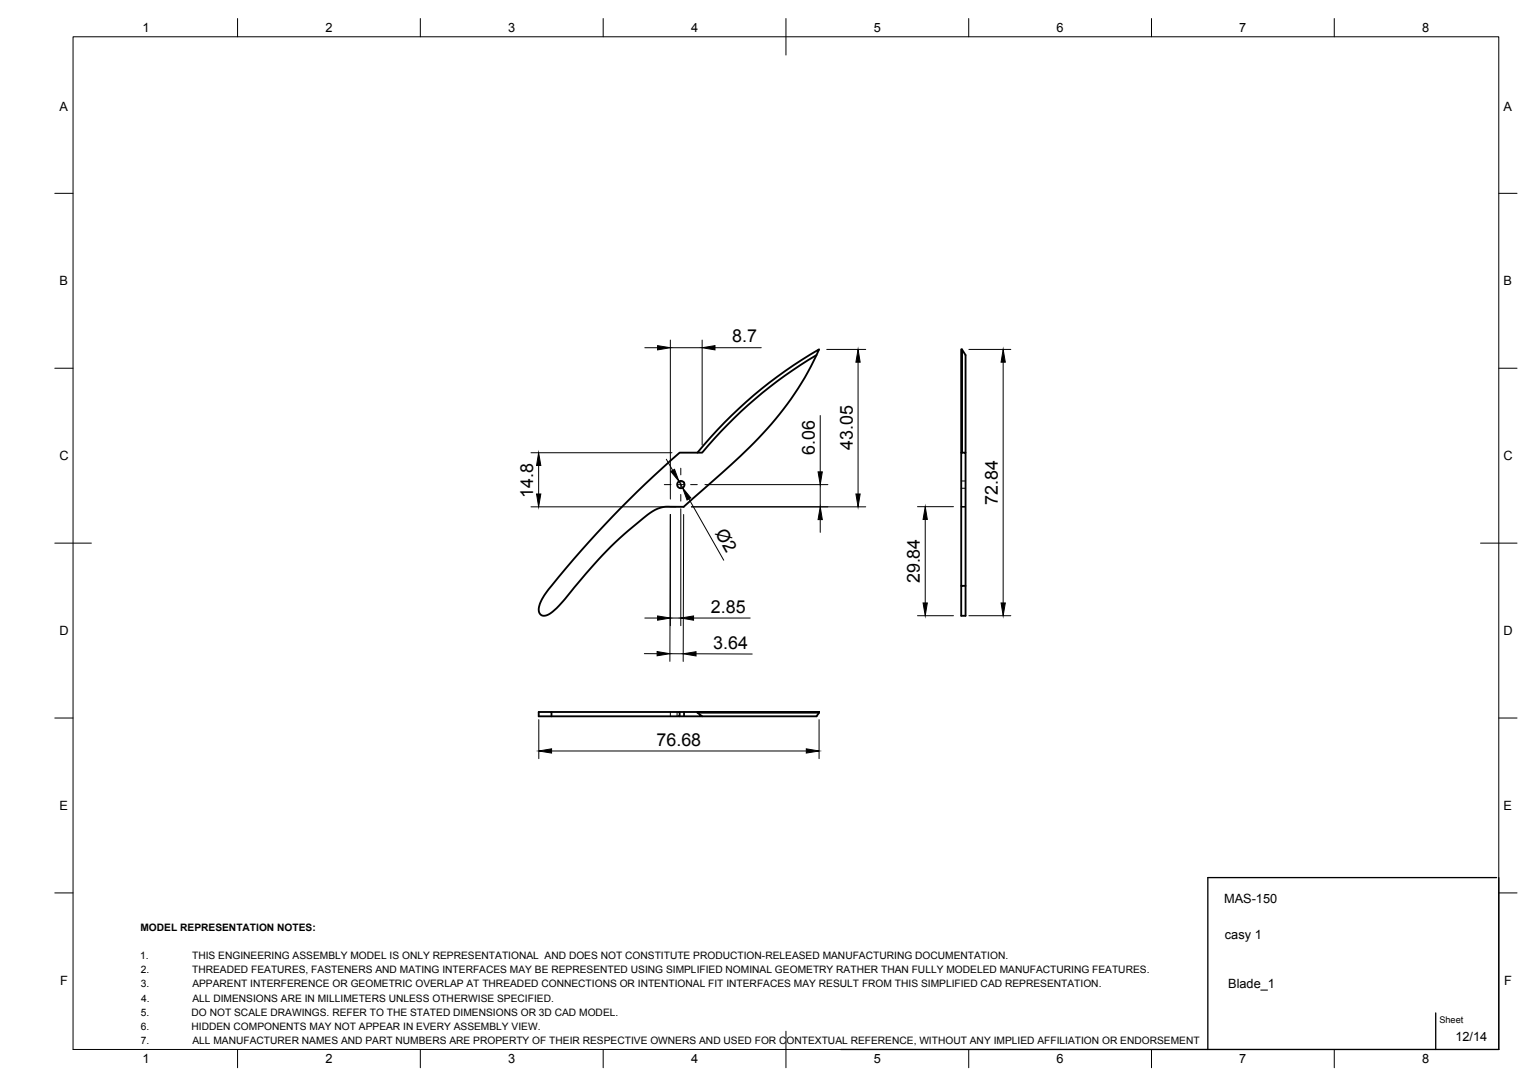
ISO-10303-21;
HEADER;
/* Generated by software containing ST-Developer
 * from STEP Tools, Inc. (www.steptools.com) 
 */

FILE_DESCRIPTION(
/* description */ ('STEP AP203'),
/* implementation_level */ '2;1');

FILE_NAME(
/* name */ 'Blade_1.step',
/* time_stamp */ '2026-11-08T21:40:52-08:00',
/* author */ (''),
/* organization */ (''),
/* preprocessor_version */ 'ST-DEVELOPER v20.2',
/* originating_system */ 'Autodesk Translation Framework v15.17.0.0',
/* authorisation */ '');

FILE_SCHEMA (('AUTOMOTIVE_DESIGN { 1 0 10303 214 3 1 1 }'));
ENDSEC;

DATA;
#10=MECHANICAL_DESIGN_GEOMETRIC_PRESENTATION_REPRESENTATION('',(#186),#12137);
#103=B_SPLINE_CURVE_WITH_KNOTS('',3,(#4610,#4611,#4612,#4613,#4614,#4615,
#4616,#4617,#4618,#4619,#4620,#4621,#4622,#4623,#4624,#4625,#4626,#4627,
#4628,#4629,#4630,#4631,#4632,#4633,#4634,#4635,#4636,#4637,#4638,#4639,
#4640,#4641,#4642,#4643,#4644,#4645,#4646,#4647,#4648,#4649,#4650,#4651,
#4652,#4653,#4654,#4655,#4656,#4657,#4658,#4659,#4660,#4661,#4662,#4663,
#4664,#4665),.UNSPECIFIED.,.F.,.F.,(4,2,2,2,2,1,2,2,2,2,2,2,2,2,2,2,2,2,
2,2,2,2,2,1,2,2,2,2,4),(1.76202838341362E-9,0.00152946839585409,0.00573422822705338,
0.00994072554036124,0.0183588914643831,0.0352156178566175,0.0520989766057049,
0.0859428491008545,0.153919387862698,0.222241646761829,0.256517065813169,
0.290860192348371,0.35972332278199,0.4287774185551,0.497967334131587,0.571128173595134,
0.636528988048645,0.709831201875327,0.774953293421917,0.843972576608793,
0.878409790177993,0.91278972931851,0.947105790641693,0.964237837412799,
0.981351495675405,0.989901182362907,0.994174197253835,0.998445976951636,
0.999999997793755),.UNSPECIFIED.);
#104=B_SPLINE_CURVE_WITH_KNOTS('',2,(#4668,#4669,#4670),.UNSPECIFIED.,.F.,
 .F.,(3,3),(0.,1.),.UNSPECIFIED.);
#105=B_SPLINE_CURVE_WITH_KNOTS('',3,(#4684,#4685,#4686,#4687,#4688,#4689,
#4690,#4691,#4692,#4693,#4694,#4695,#4696),.UNSPECIFIED.,.F.,.F.,(4,3,3,
3,4),(-0.197909908995898,-0.15516480831031,-0.111768121995836,-0.0989540665429965,
0.),.UNSPECIFIED.);
#106=B_SPLINE_CURVE_WITH_KNOTS('',3,(#4698,#4699,#4700,#4701,#4702),
 .UNSPECIFIED.,.F.,.F.,(4,1,4),(0.0298132943020683,0.494943232770503,1.),
 .UNSPECIFIED.);
#107=B_SPLINE_CURVE_WITH_KNOTS('',3,(#4705,#4706,#4707,#4708,#4709),
 .UNSPECIFIED.,.F.,.F.,(4,1,4),(0.,0.494943232770503,1.),.UNSPECIFIED.);
#108=B_SPLINE_CURVE_WITH_KNOTS('',3,(#4738,#4739,#4740,#4741,#4742,#4743,
#4744,#4745,#4746,#4747,#4748,#4749),.UNSPECIFIED.,.F.,.F.,(4,1,1,1,1,1,
1,1,1,4),(0.0654911701302355,0.0728325313021349,0.151642943092782,0.236641834545795,
0.351573197840935,0.540150564955284,0.71598472862448,0.797600110822501,
0.875509677594327,1.),.UNSPECIFIED.);
#109=B_SPLINE_CURVE_WITH_KNOTS('',3,(#4752,#4753,#4754,#4755,#4756,#4757,
#4758,#4759,#4760,#4761,#4762,#4763),.UNSPECIFIED.,.F.,.F.,(4,1,1,1,1,1,
1,1,1,4),(0.0654911701302355,0.0728325313021349,0.151642943092782,0.236641834545795,
0.351573197840935,0.540150564955284,0.71598472862448,0.797600110822501,
0.875509677594327,1.),.UNSPECIFIED.);
#110=B_SPLINE_CURVE_WITH_KNOTS('',2,(#4771,#4772,#4773),.UNSPECIFIED.,.F.,
 .F.,(3,3),(0.,1.),.UNSPECIFIED.);
#111=B_SPLINE_CURVE_WITH_KNOTS('',2,(#4776,#4777,#4778),.UNSPECIFIED.,.F.,
 .F.,(3,3),(0.,1.),.UNSPECIFIED.);
#112=B_SPLINE_CURVE_WITH_KNOTS('',3,(#4782,#4783,#4784,#4785,#4786,#4787),
 .UNSPECIFIED.,.F.,.F.,(4,2,4),(-0.229871652660954,-0.114908525875315,0.),
 .UNSPECIFIED.);
#113=B_SPLINE_CURVE_WITH_KNOTS('',3,(#4792,#4793,#4794,#4795,#4796,#4797,
#4798,#4799,#4800,#4801,#4802,#4803,#4804,#4805,#4806,#4807,#4808,#4809,
#4810,#4811,#4812,#4813,#4814,#4815,#4816,#4817,#4818,#4819,#4820,#4821,
#4822,#4823,#4824,#4825,#4826,#4827,#4828,#4829,#4830,#4831,#4832,#4833,
#4834,#4835,#4836,#4837,#4838,#4839,#4840,#4841,#4842,#4843,#4844,#4845,
#4846,#4847,#4848,#4849,#4850,#4851,#4852,#4853,#4854,#4855,#4856,#4857,
#4858),.UNSPECIFIED.,.F.,.F.,(4,3,3,3,3,3,3,3,3,3,3,3,3,3,3,3,3,3,3,3,3,
3,4),(-4.14191399419292,-4.12414475765899,-4.04926436109822,-3.89944091710028,
-3.74954461699361,-3.59958832872791,-3.29954750710329,-2.90481294303335,
-2.69931657063712,-2.30568273196656,-2.09957968336527,-2.07307122857376,
-2.04569728092775,-1.79983587858531,-1.49976903624527,-1.19950941255717,
-1.0493493530693,-0.899191607974707,-0.598950483849536,-0.298920557742038,
-0.149026588716908,-0.0741171167945361,-1.00000000280431E-6),
 .UNSPECIFIED.);
#147=B_SPLINE_SURFACE_WITH_KNOTS('',2,1,((#4600,#4601),(#4602,#4603),(#4604,
#4605)),.UNSPECIFIED.,.F.,.F.,.F.,(3,3),(2,2),(0.,1.),(0.,0.0287999999999918),
 .UNSPECIFIED.);
#148=B_SPLINE_SURFACE_WITH_KNOTS('',3,1,((#4671,#4672),(#4673,#4674),(#4675,
#4676),(#4677,#4678),(#4679,#4680),(#4681,#4682)),.UNSPECIFIED.,.F.,.F.,
 .F.,(4,1,1,4),(2,2),(0.,0.494943232770503,0.789351610361564,1.),(0.,0.17280000000419),
 .UNSPECIFIED.);
#149=B_SPLINE_SURFACE_WITH_KNOTS('',3,1,((#4710,#4711),(#4712,#4713),(#4714,
#4715),(#4716,#4717),(#4718,#4719),(#4720,#4721),(#4722,#4723),(#4724,#4725),
(#4726,#4727),(#4728,#4729),(#4730,#4731),(#4732,#4733)),.UNSPECIFIED.,
 .F.,.F.,.F.,(4,1,1,1,1,1,1,1,1,4),(2,2),(0.0654911701302355,0.0728325313021349,
0.151642943092782,0.236641834545795,0.351573197840935,0.540150564955284,
0.71598472862448,0.797600110822501,0.875509677594327,1.),(0.,0.1728),
 .UNSPECIFIED.);
#150=B_SPLINE_SURFACE_WITH_KNOTS('',2,1,((#4764,#4765),(#4766,#4767),(#4768,
#4769)),.UNSPECIFIED.,.F.,.F.,.F.,(3,3),(2,2),(0.,1.),(0.,0.1728),
 .UNSPECIFIED.);
#151=B_SPLINE_SURFACE_WITH_KNOTS('',1,3,((#4861,#4862,#4863,#4864,#4865,
#4866,#4867,#4868,#4869,#4870,#4871,#4872,#4873,#4874,#4875,#4876,#4877,
#4878,#4879,#4880,#4881,#4882,#4883,#4884,#4885,#4886,#4887,#4888,#4889,
#4890,#4891,#4892,#4893,#4894,#4895,#4896,#4897,#4898,#4899,#4900,#4901,
#4902,#4903,#4904,#4905,#4906,#4907,#4908,#4909,#4910,#4911,#4912,#4913,
#4914,#4915,#4916,#4917,#4918,#4919,#4920,#4921,#4922,#4923,#4924,#4925,
#4926,#4927,#4928,#4929,#4930,#4931,#4932,#4933,#4934,#4935,#4936,#4937,
#4938,#4939,#4940),(#4941,#4942,#4943,#4944,#4945,#4946,#4947,#4948,#4949,
#4950,#4951,#4952,#4953,#4954,#4955,#4956,#4957,#4958,#4959,#4960,#4961,
#4962,#4963,#4964,#4965,#4966,#4967,#4968,#4969,#4970,#4971,#4972,#4973,
#4974,#4975,#4976,#4977,#4978,#4979,#4980,#4981,#4982,#4983,#4984,#4985,
#4986,#4987,#4988,#4989,#4990,#4991,#4992,#4993,#4994,#4995,#4996,#4997,
#4998,#4999,#5000,#5001,#5002,#5003,#5004,#5005,#5006,#5007,#5008,#5009,
#5010,#5011,#5012,#5013,#5014,#5015,#5016,#5017,#5018,#5019,#5020)),
 .UNSPECIFIED.,.F.,.F.,.F.,(2,2),(4,2,2,2,2,2,2,2,2,2,2,2,2,2,2,2,2,2,2,
2,2,2,2,2,2,2,2,2,2,2,2,2,2,2,2,2,2,2,2,4),(0.,1.),(0.0438296453716767,
0.0445782836066419,0.0449526027241245,0.0453269218416071,0.0457012409590896,
0.0458884005178309,0.0459819802972016,0.0460755600765722,0.0462627196353135,
0.0464498791940548,0.0468241983115374,0.0475728365465026,0.0483214747814677,
0.049818751251398,0.0528133041912587,0.0558078571311194,0.0573051336010497,
0.05880241007098,0.0617969630108407,0.0647915159507014,0.067786068890562,
0.0737751747702833,0.0797642806500047,0.0827588335898653,0.0842561100597957,
0.085753386529726,0.0872506629996563,0.0879993012346215,0.0887479394695867,
0.0891222585870692,0.0893094181458105,0.0894965777045518,0.0895901574839225,
0.0896837372632931,0.0898708968220344,0.0900580563807757,0.090245215939517,
0.0906195350569996,0.0909938541744821,0.0917424924094473),.UNSPECIFIED.);
#164=SHAPE_REPRESENTATION_RELATIONSHIP('SRR','None',#12188,#175);
#175=ADVANCED_BREP_SHAPE_REPRESENTATION('',(#197),#12129);
#186=STYLED_ITEM('',(#12253),#197);
#197=MANIFOLD_SOLID_BREP('Body1',#1831);
#213=FACE_BOUND('',#648,.T.);
#214=FACE_BOUND('',#650,.T.);
#244=PLANE('',#2018);
#245=PLANE('',#2019);
#246=PLANE('',#2020);
#247=PLANE('',#2021);
#307=LINE('',#4598,#401);
#308=LINE('',#4608,#402);
#309=LINE('',#4667,#403);
#310=LINE('',#4704,#404);
#311=LINE('',#4736,#405);
#312=LINE('',#4751,#406);
#313=LINE('',#4775,#407);
#314=LINE('',#4781,#408);
#315=LINE('',#4788,#409);
#316=LINE('',#4790,#410);
#317=LINE('',#4859,#411);
#401=VECTOR('',#2303,1.);
#402=VECTOR('',#2306,1000.);
#403=VECTOR('',#2307,1000.);
#404=VECTOR('',#2308,1000.);
#405=VECTOR('',#2309,1000.);
#406=VECTOR('',#2310,1000.);
#407=VECTOR('',#2311,1000.);
#408=VECTOR('',#2314,10.);
#409=VECTOR('',#2315,10.);
#410=VECTOR('',#2318,1000.);
#411=VECTOR('',#2321,1000.);
#472=CYLINDRICAL_SURFACE('',#2015,1.);
#523=FACE_OUTER_BOUND('',#641,.T.);
#524=FACE_OUTER_BOUND('',#642,.T.);
#525=FACE_OUTER_BOUND('',#643,.T.);
#526=FACE_OUTER_BOUND('',#644,.T.);
#527=FACE_OUTER_BOUND('',#645,.T.);
#528=FACE_OUTER_BOUND('',#646,.T.);
#529=FACE_OUTER_BOUND('',#647,.T.);
#530=FACE_OUTER_BOUND('',#649,.T.);
#531=FACE_OUTER_BOUND('',#651,.T.);
#532=FACE_OUTER_BOUND('',#652,.T.);
#641=EDGE_LOOP('',(#1377,#1378,#1379,#1380));
#642=EDGE_LOOP('',(#1381,#1382,#1383,#1384));
#643=EDGE_LOOP('',(#1385,#1386,#1387,#1388,#1389));
#644=EDGE_LOOP('',(#1390,#1391,#1392,#1393));
#645=EDGE_LOOP('',(#1394,#1395,#1396,#1397));
#646=EDGE_LOOP('',(#1398,#1399,#1400,#1401,#1402));
#647=EDGE_LOOP('',(#1403,#1404,#1405,#1406,#1407,#1408));
#648=EDGE_LOOP('',(#1409));
#649=EDGE_LOOP('',(#1410,#1411,#1412,#1413,#1414,#1415));
#650=EDGE_LOOP('',(#1416));
#651=EDGE_LOOP('',(#1417,#1418,#1419,#1420));
#652=EDGE_LOOP('',(#1421,#1422,#1423,#1424));
#761=CIRCLE('',#2016,1.);
#762=CIRCLE('',#2017,1.);
#874=VERTEX_POINT('',#4595);
#875=VERTEX_POINT('',#4597);
#876=VERTEX_POINT('',#4606);
#877=VERTEX_POINT('',#4607);
#878=VERTEX_POINT('',#4609);
#879=VERTEX_POINT('',#4666);
#880=VERTEX_POINT('',#4683);
#881=VERTEX_POINT('',#4697);
#882=VERTEX_POINT('',#4703);
#883=VERTEX_POINT('',#4734);
#884=VERTEX_POINT('',#4735);
#885=VERTEX_POINT('',#4737);
#886=VERTEX_POINT('',#4750);
#887=VERTEX_POINT('',#4770);
#888=VERTEX_POINT('',#4774);
#889=VERTEX_POINT('',#4780);
#1058=EDGE_CURVE('',#874,#874,#761,.T.);
#1059=EDGE_CURVE('',#874,#875,#307,.T.);
#1060=EDGE_CURVE('',#875,#875,#762,.T.);
#1061=EDGE_CURVE('',#876,#877,#308,.T.);
#1062=EDGE_CURVE('',#877,#878,#103,.T.);
#1063=EDGE_CURVE('',#879,#878,#309,.T.);
#1064=EDGE_CURVE('',#876,#879,#104,.T.);
#1065=EDGE_CURVE('',#878,#880,#105,.T.);
#1066=EDGE_CURVE('',#880,#881,#106,.T.);
#1067=EDGE_CURVE('',#882,#881,#310,.T.);
#1068=EDGE_CURVE('',#879,#882,#107,.T.);
#1069=EDGE_CURVE('',#883,#884,#311,.T.);
#1070=EDGE_CURVE('',#885,#883,#108,.T.);
#1071=EDGE_CURVE('',#885,#886,#312,.T.);
#1072=EDGE_CURVE('',#886,#884,#109,.T.);
#1073=EDGE_CURVE('',#884,#887,#110,.T.);
#1074=EDGE_CURVE('',#888,#887,#313,.T.);
#1075=EDGE_CURVE('',#883,#888,#111,.T.);
#1076=EDGE_CURVE('',#887,#889,#314,.T.);
#1077=EDGE_CURVE('',#889,#877,#112,.T.);
#1078=EDGE_CURVE('',#888,#876,#315,.T.);
#1079=EDGE_CURVE('',#885,#882,#316,.T.);
#1080=EDGE_CURVE('',#880,#889,#113,.T.);
#1081=EDGE_CURVE('',#881,#886,#317,.T.);
#1377=ORIENTED_EDGE('',*,*,#1058,.F.);
#1378=ORIENTED_EDGE('',*,*,#1059,.T.);
#1379=ORIENTED_EDGE('',*,*,#1060,.T.);
#1380=ORIENTED_EDGE('',*,*,#1059,.F.);
#1381=ORIENTED_EDGE('',*,*,#1061,.T.);
#1382=ORIENTED_EDGE('',*,*,#1062,.T.);
#1383=ORIENTED_EDGE('',*,*,#1063,.F.);
#1384=ORIENTED_EDGE('',*,*,#1064,.F.);
#1385=ORIENTED_EDGE('',*,*,#1063,.T.);
#1386=ORIENTED_EDGE('',*,*,#1065,.T.);
#1387=ORIENTED_EDGE('',*,*,#1066,.T.);
#1388=ORIENTED_EDGE('',*,*,#1067,.F.);
#1389=ORIENTED_EDGE('',*,*,#1068,.F.);
#1390=ORIENTED_EDGE('',*,*,#1069,.F.);
#1391=ORIENTED_EDGE('',*,*,#1070,.F.);
#1392=ORIENTED_EDGE('',*,*,#1071,.T.);
#1393=ORIENTED_EDGE('',*,*,#1072,.T.);
#1394=ORIENTED_EDGE('',*,*,#1073,.T.);
#1395=ORIENTED_EDGE('',*,*,#1074,.F.);
#1396=ORIENTED_EDGE('',*,*,#1075,.F.);
#1397=ORIENTED_EDGE('',*,*,#1069,.T.);
#1398=ORIENTED_EDGE('',*,*,#1076,.T.);
#1399=ORIENTED_EDGE('',*,*,#1077,.T.);
#1400=ORIENTED_EDGE('',*,*,#1061,.F.);
#1401=ORIENTED_EDGE('',*,*,#1078,.F.);
#1402=ORIENTED_EDGE('',*,*,#1074,.T.);
#1403=ORIENTED_EDGE('',*,*,#1068,.T.);
#1404=ORIENTED_EDGE('',*,*,#1079,.F.);
#1405=ORIENTED_EDGE('',*,*,#1070,.T.);
#1406=ORIENTED_EDGE('',*,*,#1075,.T.);
#1407=ORIENTED_EDGE('',*,*,#1078,.T.);
#1408=ORIENTED_EDGE('',*,*,#1064,.T.);
#1409=ORIENTED_EDGE('',*,*,#1060,.F.);
#1410=ORIENTED_EDGE('',*,*,#1066,.F.);
#1411=ORIENTED_EDGE('',*,*,#1080,.T.);
#1412=ORIENTED_EDGE('',*,*,#1076,.F.);
#1413=ORIENTED_EDGE('',*,*,#1073,.F.);
#1414=ORIENTED_EDGE('',*,*,#1072,.F.);
#1415=ORIENTED_EDGE('',*,*,#1081,.F.);
#1416=ORIENTED_EDGE('',*,*,#1058,.T.);
#1417=ORIENTED_EDGE('',*,*,#1079,.T.);
#1418=ORIENTED_EDGE('',*,*,#1067,.T.);
#1419=ORIENTED_EDGE('',*,*,#1081,.T.);
#1420=ORIENTED_EDGE('',*,*,#1071,.F.);
#1421=ORIENTED_EDGE('',*,*,#1077,.F.);
#1422=ORIENTED_EDGE('',*,*,#1080,.F.);
#1423=ORIENTED_EDGE('',*,*,#1065,.F.);
#1424=ORIENTED_EDGE('',*,*,#1062,.F.);
#1751=ADVANCED_FACE('',(#523),#472,.F.);
#1752=ADVANCED_FACE('',(#524),#147,.F.);
#1753=ADVANCED_FACE('',(#525),#148,.F.);
#1754=ADVANCED_FACE('',(#526),#149,.F.);
#1755=ADVANCED_FACE('',(#527),#150,.F.);
#1756=ADVANCED_FACE('',(#528),#244,.F.);
#1757=ADVANCED_FACE('',(#529,#213),#245,.F.);
#1758=ADVANCED_FACE('',(#530,#214),#246,.T.);
#1759=ADVANCED_FACE('',(#531),#247,.F.);
#1760=ADVANCED_FACE('',(#532),#151,.T.);
#1831=CLOSED_SHELL('',(#1751,#1752,#1753,#1754,#1755,#1756,#1757,#1758,
#1759,#1760));
#2014=AXIS2_PLACEMENT_3D('',#4593,#2297,#2298);
#2015=AXIS2_PLACEMENT_3D('',#4594,#2299,#2300);
#2016=AXIS2_PLACEMENT_3D('',#4596,#2301,#2302);
#2017=AXIS2_PLACEMENT_3D('',#4599,#2304,#2305);
#2018=AXIS2_PLACEMENT_3D('',#4779,#2312,#2313);
#2019=AXIS2_PLACEMENT_3D('',#4789,#2316,#2317);
#2020=AXIS2_PLACEMENT_3D('',#4791,#2319,#2320);
#2021=AXIS2_PLACEMENT_3D('',#4860,#2322,#2323);
#2297=DIRECTION('axis',(0.,0.,1.));
#2298=DIRECTION('refdir',(1.,0.,0.));
#2299=DIRECTION('center_axis',(0.,1.,0.));
#2300=DIRECTION('ref_axis',(1.11022302462515E-16,0.,1.));
#2301=DIRECTION('center_axis',(0.,1.,0.));
#2302=DIRECTION('ref_axis',(1.11022302462515E-16,0.,1.));
#2303=DIRECTION('',(0.,1.,0.));
#2304=DIRECTION('center_axis',(0.,1.,0.));
#2305=DIRECTION('ref_axis',(1.11022302462515E-16,0.,1.));
#2306=DIRECTION('',(0.,-1.,0.));
#2307=DIRECTION('',(0.,-1.,0.));
#2308=DIRECTION('',(0.,-1.,0.));
#2309=DIRECTION('',(0.,-1.,0.));
#2310=DIRECTION('',(0.,-1.,0.));
#2311=DIRECTION('',(0.,-1.,0.));
#2312=DIRECTION('center_axis',(0.318513611714452,0.,0.94791828717069));
#2313=DIRECTION('ref_axis',(0.94791828717069,0.,-0.318513611714452));
#2314=DIRECTION('',(-0.94791828717069,0.,0.318513611714452));
#2315=DIRECTION('',(-0.947918287170691,0.,0.318513611714451));
#2316=DIRECTION('center_axis',(0.,-1.,0.));
#2317=DIRECTION('ref_axis',(-1.11022302462515E-16,0.,-1.));
#2318=DIRECTION('',(-0.946888830122557,0.,0.321561103663262));
#2319=DIRECTION('center_axis',(0.,-1.,0.));
#2320=DIRECTION('ref_axis',(-1.11022302462515E-16,0.,-1.));
#2321=DIRECTION('',(0.946888830122557,0.,-0.321561103663262));
#2322=DIRECTION('center_axis',(-0.321561103663262,0.,-0.946888830122557));
#2323=DIRECTION('ref_axis',(-0.946888830122557,0.,0.321561103663262));
#4593=CARTESIAN_POINT('',(0.,0.,0.));
#4594=CARTESIAN_POINT('Origin',(0.,0.,-0.451382872428838));
#4595=CARTESIAN_POINT('',(-2.33486982377251E-16,0.,-1.45138287242884));
#4596=CARTESIAN_POINT('Origin',(0.,0.,-0.451382872428838));
#4597=CARTESIAN_POINT('',(-2.33486982377251E-16,1.2,-1.45138287242884));
#4598=CARTESIAN_POINT('',(-2.3348698237725E-16,0.,-1.45138287242884));
#4599=CARTESIAN_POINT('Origin',(0.,1.2,-0.451382872428838));
#4600=CARTESIAN_POINT('Ctrl Pts',(-7.09134809128677,1.2,-7.28017474573539));
#4601=CARTESIAN_POINT('Ctrl Pts',(-7.09134809128677,0.912000000000082,-7.28017474573539));
#4602=CARTESIAN_POINT('Ctrl Pts',(-26.0573343465012,1.2,-19.1299473575062));
#4603=CARTESIAN_POINT('Ctrl Pts',(-26.0573343465012,0.912000000000082,-19.1299473575062));
#4604=CARTESIAN_POINT('Ctrl Pts',(-47.6352267379569,1.2,-23.4630266781973));
#4605=CARTESIAN_POINT('Ctrl Pts',(-47.6352267379569,0.912000000000082,-23.4630266781973));
#4606=CARTESIAN_POINT('',(-7.09134809128677,1.2,-7.28017474573539));
#4607=CARTESIAN_POINT('',(-7.09134823816015,1.00000000000006,-7.28017467283774));
#4608=CARTESIAN_POINT('',(-7.09134809128677,1.2,-7.28017474573539));
#4609=CARTESIAN_POINT('',(-47.6352266725888,1.00000007481202,-23.463026510487));
#4610=CARTESIAN_POINT('Ctrl Pts',(-7.09134831553042,1.00000000000006,-7.28017453553405));
#4611=CARTESIAN_POINT('Ctrl Pts',(-7.11068751337854,1.00000000000006,-7.29225607297566));
#4612=CARTESIAN_POINT('Ctrl Pts',(-7.13014127538947,1.00000000000006,-7.3044055075262));
#4613=CARTESIAN_POINT('Ctrl Pts',(-7.20288303224859,1.00000000000006,-7.34979888829056));
#4614=CARTESIAN_POINT('Ctrl Pts',(-7.2562856468552,1.00000000000006,-7.38307141655157));
#4615=CARTESIAN_POINT('Ctrl Pts',(-7.36308604485071,1.00000000000006,-7.44950314916467));
#4616=CARTESIAN_POINT('Ctrl Pts',(-7.41650933220709,1.00000000000006,-7.48267908965507));
#4617=CARTESIAN_POINT('Ctrl Pts',(-7.57688126501097,1.00000000000006,-7.58210746819504));
#4618=CARTESIAN_POINT('Ctrl Pts',(-7.68386634925554,1.00000000000006,-7.64821950621151));
#4619=CARTESIAN_POINT('Ctrl Pts',(-8.00522827087396,1.00000000000006,-7.84615547748184));
#4620=CARTESIAN_POINT('Ctrl Pts',(-8.43461654073609,1.00000000000006,-8.10888740557686));
#4621=CARTESIAN_POINT('Ctrl Pts',(-8.86481189078967,1.00000000000006,-8.36863733500345));
#4622=CARTESIAN_POINT('Ctrl Pts',(-9.51221899491459,1.00000000000005,-8.75693190854638));
#4623=CARTESIAN_POINT('Ctrl Pts',(-9.94498238629759,1.00000000000006,-9.01300707260298));
#4624=CARTESIAN_POINT('Ctrl Pts',(-11.2495773841444,1.00000000000006,-9.77452717708374));
#4625=CARTESIAN_POINT('Ctrl Pts',(-12.1240421591257,1.00000000000006,-10.2710077251322));
#4626=CARTESIAN_POINT('Ctrl Pts',(-13.8850801361361,1.00000000000006,-11.2430286125482));
#4627=CARTESIAN_POINT('Ctrl Pts',(-14.7716680498301,1.00000000000006,-11.7184360575102));
#4628=CARTESIAN_POINT('Ctrl Pts',(-16.1094164672201,1.00000000000006,-12.4149117109426));
#4629=CARTESIAN_POINT('Ctrl Pts',(-16.5574356159811,1.00000000000006,-12.6446827728682));
#4630=CARTESIAN_POINT('Ctrl Pts',(-17.4559246536095,1.00000000000006,-13.0985360950426));
#4631=CARTESIAN_POINT('Ctrl Pts',(-17.906495383924,1.00000000000006,-13.3226581958257));
#4632=CARTESIAN_POINT('Ctrl Pts',(-19.2630950583786,1.00000000000006,-13.9870499958456));
#4633=CARTESIAN_POINT('Ctrl Pts',(-20.1719150319432,1.00000000000006,-14.4182572383939));
#4634=CARTESIAN_POINT('Ctrl Pts',(-21.9998979114302,1.00000000000006,-15.2579388305516));
#4635=CARTESIAN_POINT('Ctrl Pts',(-22.9191119697774,1.00000000000006,-15.6663622503542));
#4636=CARTESIAN_POINT('Ctrl Pts',(-24.768006788053,1.00000000000006,-16.4603187472532));
#4637=CARTESIAN_POINT('Ctrl Pts',(-25.6976797513383,1.00000000000006,-16.8457952774682));
#4638=CARTESIAN_POINT('Ctrl Pts',(-27.620212900096,1.00000000000006,-17.6147290858774));
#4639=CARTESIAN_POINT('Ctrl Pts',(-28.6120762515168,1.00000000000006,-17.9961739561557));
#4640=CARTESIAN_POINT('Ctrl Pts',(-30.4984832918179,1.00000000000006,-18.6929702060858));
#4641=CARTESIAN_POINT('Ctrl Pts',(-31.3921908423818,1.00000000000006,-19.0110399067431));
#4642=CARTESIAN_POINT('Ctrl Pts',(-33.2952368599222,1.00000000000006,-19.6629165069278));
#4643=CARTESIAN_POINT('Ctrl Pts',(-34.3055473016782,1.00000000000006,-19.9939988746763));
#4644=CARTESIAN_POINT('Ctrl Pts',(-36.2228941614421,1.00000000000006,-20.5941180293612));
#4645=CARTESIAN_POINT('Ctrl Pts',(-37.1288738936713,1.00000000000006,-20.8659549929327));
#4646=CARTESIAN_POINT('Ctrl Pts',(-39.003851405174,1.00000000000006,-21.4044110917491));
#4647=CARTESIAN_POINT('Ctrl Pts',(-39.9735095225768,1.00000000000006,-21.6697762014278));
#4648=CARTESIAN_POINT('Ctrl Pts',(-41.4346591386383,1.00000000000006,-22.0500145741695));
#4649=CARTESIAN_POINT('Ctrl Pts',(-41.9223778391297,1.00000000000006,-22.1736882842118));
#4650=CARTESIAN_POINT('Ctrl Pts',(-42.8996532716617,1.00000000000006,-22.4150132014848));
#4651=CARTESIAN_POINT('Ctrl Pts',(-43.3893152843367,1.00000000000006,-22.5326978063825));
#4652=CARTESIAN_POINT('Ctrl Pts',(-44.3696193969244,1.00000000000006,-22.7618534517681));
#4653=CARTESIAN_POINT('Ctrl Pts',(-44.8604283639025,1.00000000000006,-22.8733785049591));
#4654=CARTESIAN_POINT('Ctrl Pts',(-45.5979342111895,1.00000000000006,-23.0361575203374));
#4655=CARTESIAN_POINT('Ctrl Pts',(-46.0894060993012,1.00000000000006,-23.1430409487816));
#4656=CARTESIAN_POINT('Ctrl Pts',(-46.5820249421721,1.00000000000006,-23.2469929425543));
#4657=CARTESIAN_POINT('Ctrl Pts',(-46.951626660381,1.00000000000006,-23.3237965794452));
#4658=CARTESIAN_POINT('Ctrl Pts',(-47.074831674522,1.00000000000006,-23.34920099103));
#4659=CARTESIAN_POINT('Ctrl Pts',(-47.2597235085411,1.00000000000006,-23.3870284915049));
#4660=CARTESIAN_POINT('Ctrl Pts',(-47.3213549739448,1.00000000000006,-23.3995884807167));
#4661=CARTESIAN_POINT('Ctrl Pts',(-47.4446371365223,1.00000000000006,-23.4246136938071));
#4662=CARTESIAN_POINT('Ctrl Pts',(-47.5063193313214,1.00000000000006,-23.4370845030402));
#4663=CARTESIAN_POINT('Ctrl Pts',(-47.5903801898929,1.00000000000006,-23.4540147689754));
#4664=CARTESIAN_POINT('Ctrl Pts',(-47.6128719552537,1.00000000000006,-23.4585359892155));
#4665=CARTESIAN_POINT('Ctrl Pts',(-47.6352267041176,1.00000000000006,-23.4630263535246));
#4666=CARTESIAN_POINT('',(-47.6352267379569,1.2,-23.4630266781973));
#4667=CARTESIAN_POINT('',(-47.6352267379569,1.2,-23.4630266781973));
#4668=CARTESIAN_POINT('Ctrl Pts',(-7.09134809128677,1.2,-7.28017474573539));
#4669=CARTESIAN_POINT('Ctrl Pts',(-26.0573343465012,1.2,-19.1299473575062));
#4670=CARTESIAN_POINT('Ctrl Pts',(-47.6352267379569,1.2,-23.4630266781973));
#4671=CARTESIAN_POINT('Ctrl Pts',(-47.6352267379569,1.2,-23.4630266781973));
#4672=CARTESIAN_POINT('Ctrl Pts',(-47.6352267379569,-0.5280000000419,-23.4630266781973));
#4673=CARTESIAN_POINT('Ctrl Pts',(-41.2879795894165,1.2,-16.3973366595173));
#4674=CARTESIAN_POINT('Ctrl Pts',(-41.2879795894165,-0.5280000000419,-16.3973366595173));
#4675=CARTESIAN_POINT('Ctrl Pts',(-28.9390638541746,1.2,-7.40052527015664));
#4676=CARTESIAN_POINT('Ctrl Pts',(-28.9390638541746,-0.5280000000419,-7.40052527015664));
#4677=CARTESIAN_POINT('Ctrl Pts',(-11.4361348672924,1.2,0.292821829763132));
#4678=CARTESIAN_POINT('Ctrl Pts',(-11.4361348672924,-0.5280000000419,0.292821829763132));
#4679=CARTESIAN_POINT('Ctrl Pts',(-2.50014102937161,1.2,3.94559933269074));
#4680=CARTESIAN_POINT('Ctrl Pts',(-2.50014102937161,-0.5280000000419,3.94559933269074));
#4681=CARTESIAN_POINT('Ctrl Pts',(1.18077271965353,1.2,5.54861712757117));
#4682=CARTESIAN_POINT('Ctrl Pts',(1.18077271965353,-0.5280000000419,5.54861712757117));
#4683=CARTESIAN_POINT('',(-46.4732177923012,0.,-22.2016498092846));
#4684=CARTESIAN_POINT('Ctrl Pts',(-47.6352265853192,1.00000017512283,-23.4630265082826));
#4685=CARTESIAN_POINT('Ctrl Pts',(-47.5497337833158,0.923530724722877,-23.3678568040681));
#4686=CARTESIAN_POINT('Ctrl Pts',(-47.4664431491314,0.849654487371893,-23.275672245252));
#4687=CARTESIAN_POINT('Ctrl Pts',(-47.3838551040137,0.777007709588356,-23.1847477783321));
#4688=CARTESIAN_POINT('Ctrl Pts',(-47.3000081267036,0.7032535394808,-23.0924373028402));
#4689=CARTESIAN_POINT('Ctrl Pts',(-47.2168852312997,0.630766597197125,-23.0014256885189));
#4690=CARTESIAN_POINT('Ctrl Pts',(-47.1328800183873,0.558119808566171,-22.9099457634324));
#4691=CARTESIAN_POINT('Ctrl Pts',(-47.1080751876962,0.536668862490658,-22.8829338200692));
#4692=CARTESIAN_POINT('Ctrl Pts',(-47.0831931883918,0.515203979624482,-22.8558812926668));
#4693=CARTESIAN_POINT('Ctrl Pts',(-47.0581920598092,0.493688420180458,-22.8287433089684));
#4694=CARTESIAN_POINT('Ctrl Pts',(-46.8651256765308,0.327538670886058,-22.6191754750683));
#4695=CARTESIAN_POINT('Ctrl Pts',(-46.6701360902887,0.162956146341853,-22.4101382936785));
#4696=CARTESIAN_POINT('Ctrl Pts',(-46.4732177923012,0.,-22.2016498092846));
#4697=CARTESIAN_POINT('',(1.18077271965353,0.,5.54861712757117));
#4698=CARTESIAN_POINT('Ctrl Pts',(-46.4732177923012,0.,-22.2016498092846));
#4699=CARTESIAN_POINT('Ctrl Pts',(-40.3530658599041,0.,-15.7219005239919));
#4700=CARTESIAN_POINT('Ctrl Pts',(-25.1069939231375,0.,-4.7997213617563));
#4701=CARTESIAN_POINT('Ctrl Pts',(-7.64469421946831,0.,1.70517457060066));
#4702=CARTESIAN_POINT('Ctrl Pts',(1.18077271965353,0.,5.54861712757117));
#4703=CARTESIAN_POINT('',(1.18077271965353,1.2,5.54861712757117));
#4704=CARTESIAN_POINT('',(1.18077271965353,1.2,5.54861712757117));
#4705=CARTESIAN_POINT('Ctrl Pts',(-47.6352267379569,1.2,-23.4630266781973));
#4706=CARTESIAN_POINT('Ctrl Pts',(-41.2879795894165,1.2,-16.3973366595173));
#4707=CARTESIAN_POINT('Ctrl Pts',(-25.6436006166727,1.2,-4.99961317195811));
#4708=CARTESIAN_POINT('Ctrl Pts',(-7.64469421946831,1.2,1.70517457060066));
#4709=CARTESIAN_POINT('Ctrl Pts',(1.18077271965353,1.2,5.54861712757117));
#4710=CARTESIAN_POINT('Ctrl Pts',(4.63072594339218,1.2,4.37702154953648));
#4711=CARTESIAN_POINT('Ctrl Pts',(4.63072594339218,-0.528,4.37702154953648));
#4712=CARTESIAN_POINT('Ctrl Pts',(4.7840847941358,1.2,4.31192383490808));
#4713=CARTESIAN_POINT('Ctrl Pts',(4.7840847941358,-0.528,4.31192383490808));
#4714=CARTESIAN_POINT('Ctrl Pts',(6.57703737715603,1.2,3.59239489692552));
#4715=CARTESIAN_POINT('Ctrl Pts',(6.57703737715603,-0.528,3.59239489692552));
#4716=CARTESIAN_POINT('Ctrl Pts',(9.67706435206833,1.2,3.76607425470487));
#4717=CARTESIAN_POINT('Ctrl Pts',(9.67706435206833,-0.528,3.76607425470487));
#4718=CARTESIAN_POINT('Ctrl Pts',(14.6739773919611,1.2,5.78899007926008));
#4719=CARTESIAN_POINT('Ctrl Pts',(14.6739773919611,-0.528,5.78899007926008));
#4720=CARTESIAN_POINT('Ctrl Pts',(21.529136784602,1.2,8.35971201308491));
#4721=CARTESIAN_POINT('Ctrl Pts',(21.529136784602,-0.528,8.35971201308491));
#4722=CARTESIAN_POINT('Ctrl Pts',(29.5112752479747,1.2,12.6039811673409));
#4723=CARTESIAN_POINT('Ctrl Pts',(29.5112752479747,-0.528,12.6039811673409));
#4724=CARTESIAN_POINT('Ctrl Pts',(36.9335047542113,1.2,17.1028493432964));
#4725=CARTESIAN_POINT('Ctrl Pts',(36.9335047542113,-0.528,17.1028493432964));
#4726=CARTESIAN_POINT('Ctrl Pts',(41.8538494170237,1.2,20.3434433890621));
#4727=CARTESIAN_POINT('Ctrl Pts',(41.8538494170237,-0.528,20.3434433890621));
#4728=CARTESIAN_POINT('Ctrl Pts',(48.2654669907203,1.2,23.135880733102));
#4729=CARTESIAN_POINT('Ctrl Pts',(48.2654669907203,-0.528,23.135880733102));
#4730=CARTESIAN_POINT('Ctrl Pts',(48.9333109271159,1.2,18.4504184980571));
#4731=CARTESIAN_POINT('Ctrl Pts',(48.9333109271159,-0.528,18.4504184980571));
#4732=CARTESIAN_POINT('Ctrl Pts',(42.3375494192901,1.2,14.5257061310277));
#4733=CARTESIAN_POINT('Ctrl Pts',(42.3375494192901,-0.528,14.5257061310277));
#4734=CARTESIAN_POINT('',(42.3375494192901,1.2,14.5257061310277));
#4735=CARTESIAN_POINT('',(42.3375494192901,0.,14.5257061310277));
#4736=CARTESIAN_POINT('',(42.3375494192901,1.2,14.5257061310277));
#4737=CARTESIAN_POINT('',(4.63072594277028,1.2,4.37702154980046));
#4738=CARTESIAN_POINT('Ctrl Pts',(4.63072594339218,1.2,4.37702154953648));
#4739=CARTESIAN_POINT('Ctrl Pts',(4.7840847941358,1.2,4.31192383490808));
#4740=CARTESIAN_POINT('Ctrl Pts',(6.57703737715603,1.2,3.59239489692552));
#4741=CARTESIAN_POINT('Ctrl Pts',(9.67706435206833,1.2,3.76607425470487));
#4742=CARTESIAN_POINT('Ctrl Pts',(14.6739773919611,1.2,5.78899007926008));
#4743=CARTESIAN_POINT('Ctrl Pts',(21.529136784602,1.2,8.35971201308491));
#4744=CARTESIAN_POINT('Ctrl Pts',(29.5112752479747,1.2,12.6039811673409));
#4745=CARTESIAN_POINT('Ctrl Pts',(36.9335047542113,1.2,17.1028493432964));
#4746=CARTESIAN_POINT('Ctrl Pts',(41.8538494170237,1.2,20.3434433890621));
#4747=CARTESIAN_POINT('Ctrl Pts',(48.2654669907203,1.2,23.135880733102));
#4748=CARTESIAN_POINT('Ctrl Pts',(48.9333109271159,1.2,18.4504184980571));
#4749=CARTESIAN_POINT('Ctrl Pts',(42.3375494192901,1.2,14.5257061310277));
#4750=CARTESIAN_POINT('',(4.63072594277028,0.,4.37702154980046));
#4751=CARTESIAN_POINT('',(4.63072594277027,1.2,4.37702154980048));
#4752=CARTESIAN_POINT('Ctrl Pts',(4.63072594339218,4.16333634234434E-16,
4.37702154953648));
#4753=CARTESIAN_POINT('Ctrl Pts',(4.7840847941358,4.16333634234434E-16,
4.31192383490808));
#4754=CARTESIAN_POINT('Ctrl Pts',(6.57703737715603,4.16333634234434E-16,
3.59239489692552));
#4755=CARTESIAN_POINT('Ctrl Pts',(9.67706435206833,4.16333634234434E-16,
3.76607425470487));
#4756=CARTESIAN_POINT('Ctrl Pts',(14.6739773919611,4.16333634234434E-16,
5.78899007926008));
#4757=CARTESIAN_POINT('Ctrl Pts',(21.529136784602,4.16333634234434E-16,
8.35971201308491));
#4758=CARTESIAN_POINT('Ctrl Pts',(29.5112752479747,4.16333634234434E-16,
12.6039811673409));
#4759=CARTESIAN_POINT('Ctrl Pts',(36.9335047542113,4.16333634234434E-16,
17.1028493432964));
#4760=CARTESIAN_POINT('Ctrl Pts',(41.8538494170237,4.16333634234434E-16,
20.3434433890621));
#4761=CARTESIAN_POINT('Ctrl Pts',(48.2654669907203,4.16333634234434E-16,
23.135880733102));
#4762=CARTESIAN_POINT('Ctrl Pts',(48.9333109271159,4.16333634234434E-16,
18.4504184980571));
#4763=CARTESIAN_POINT('Ctrl Pts',(42.3375494192901,4.16333634234434E-16,
14.5257061310277));
#4764=CARTESIAN_POINT('Ctrl Pts',(42.3375494192901,1.2,14.5257061310277));
#4765=CARTESIAN_POINT('Ctrl Pts',(42.3375494192901,-0.528,14.5257061310277));
#4766=CARTESIAN_POINT('Ctrl Pts',(20.9640318338388,1.2,0.869135776253969));
#4767=CARTESIAN_POINT('Ctrl Pts',(20.9640318338388,-0.528,0.869135776253969));
#4768=CARTESIAN_POINT('Ctrl Pts',(-2.47626210225015,1.2,-8.83090725784708));
#4769=CARTESIAN_POINT('Ctrl Pts',(-2.47626210225015,-0.528,-8.83090725784708));
#4770=CARTESIAN_POINT('',(-2.47626210225015,0.,-8.83090725784708));
#4771=CARTESIAN_POINT('Ctrl Pts',(42.3375494192901,0.,14.5257061310277));
#4772=CARTESIAN_POINT('Ctrl Pts',(20.9640318338388,0.,0.869135776253969));
#4773=CARTESIAN_POINT('Ctrl Pts',(-2.47626210225015,0.,-8.83090725784708));
#4774=CARTESIAN_POINT('',(-2.47626210225015,1.2,-8.83090725784708));
#4775=CARTESIAN_POINT('',(-2.47626210225015,1.2,-8.83090725784708));
#4776=CARTESIAN_POINT('Ctrl Pts',(42.3375494192901,1.2,14.5257061310277));
#4777=CARTESIAN_POINT('Ctrl Pts',(20.9640318338388,1.2,0.869135776253969));
#4778=CARTESIAN_POINT('Ctrl Pts',(-2.47626210225015,1.2,-8.83090725784708));
#4779=CARTESIAN_POINT('Origin',(-2.47626210225015,1.2,-8.83090725784708));
#4780=CARTESIAN_POINT('',(-8.32185266851751,0.,-6.86670824505761));
#4781=CARTESIAN_POINT('',(-2.47626210225015,0.,-8.83090725784708));
#4782=CARTESIAN_POINT('Ctrl Pts',(-8.32185266851834,1.14311338172968E-12,
-6.86670824505734));
#4783=CARTESIAN_POINT('Ctrl Pts',(-8.11928072190117,0.164182972460768,-6.93477521161165));
#4784=CARTESIAN_POINT('Ctrl Pts',(-7.91680514284801,0.328508227719272,-7.00280979716715));
#4785=CARTESIAN_POINT('Ctrl Pts',(-7.51215815602449,0.657345458539218,-7.13877676287178));
#4786=CARTESIAN_POINT('Ctrl Pts',(-7.37869817804401,0.765866874721603,-7.18362115541202));
#4787=CARTESIAN_POINT('Ctrl Pts',(-7.09134844131163,1.00000001188238,-7.28017462812221));
#4788=CARTESIAN_POINT('',(-2.47626210225015,1.2,-8.83090725784708));
#4789=CARTESIAN_POINT('Origin',(-26.7103108805615,1.2,-17.2507740347362));
#4790=CARTESIAN_POINT('',(1.18077271965353,1.2,5.54861712757117));
#4791=CARTESIAN_POINT('Origin',(-26.7103108805615,0.,-17.2507740347362));
#4792=CARTESIAN_POINT('Ctrl Pts',(-46.4732177922936,0.,-22.2016498093203));
#4793=CARTESIAN_POINT('Ctrl Pts',(-46.415282761538,5.07841822769624E-16,
-22.1893264214989));
#4794=CARTESIAN_POINT('Ctrl Pts',(-46.3573586444288,1.28814513242496E-15,
-22.176961010912));
#4795=CARTESIAN_POINT('Ctrl Pts',(-46.2994454089906,1.77635683940025E-15,
-22.1645535547065));
#4796=CARTESIAN_POINT('Ctrl Pts',(-46.0553963173232,3.8337038815267E-15,
-22.1122679520467));
#4797=CARTESIAN_POINT('Ctrl Pts',(-45.8115404634548,5.56211880942695E-15,
-22.0592357000739));
#4798=CARTESIAN_POINT('Ctrl Pts',(-45.5678754638484,7.32747196252603E-15,
-22.0054550434754));
#4799=CARTESIAN_POINT('Ctrl Pts',(-45.0803415951789,1.08596553031322E-14,
-21.8978487331172));
#4800=CARTESIAN_POINT('Ctrl Pts',(-44.5935547144433,1.37433652042168E-14,
-21.7872420837894));
#4801=CARTESIAN_POINT('Ctrl Pts',(-44.1075470623437,1.62092561595273E-14,
-21.6736330559672));
#4802=CARTESIAN_POINT('Ctrl Pts',(-43.6213030745586,1.86763462277054E-14,
-21.559968782374));
#4803=CARTESIAN_POINT('Ctrl Pts',(-43.1356693881152,2.06773659315811E-14,
-21.443256509246));
#4804=CARTESIAN_POINT('Ctrl Pts',(-42.65115708627,2.26485497023532E-14,
-21.3236127657438));
#4805=CARTESIAN_POINT('Ctrl Pts',(-42.1664508837015,2.46205223363956E-14,
-21.2039211410871));
#4806=CARTESIAN_POINT('Ctrl Pts',(-41.6827582533232,2.48053267803675E-14,
-21.0812721899324));
#4807=CARTESIAN_POINT('Ctrl Pts',(-41.2001345714453,2.62012633811537E-14,
-20.9556779035789));
#4808=CARTESIAN_POINT('Ctrl Pts',(-40.2344744599496,2.87722289092885E-14,
-20.7043819205649));
#4809=CARTESIAN_POINT('Ctrl Pts',(-39.2727950142657,2.70692054571062E-14,
-20.4412269998355));
#4810=CARTESIAN_POINT('Ctrl Pts',(-38.3151477577178,2.62012633811537E-14,
-20.1662098332526));
#4811=CARTESIAN_POINT('Ctrl Pts',(-37.0552642848644,2.50593963007545E-14,
-19.8043964614086));
#4812=CARTESIAN_POINT('Ctrl Pts',(-35.8021293334856,2.23739275243883E-14,
-19.4219998183265));
#4813=CARTESIAN_POINT('Ctrl Pts',(-34.5554354702551,1.95399252334028E-14,
-19.018867339076));
#4814=CARTESIAN_POINT('Ctrl Pts',(-33.9064143565704,1.80645611706375E-14,
-18.8089990639827));
#4815=CARTESIAN_POINT('Ctrl Pts',(-33.2591391506989,1.64907532665174E-14,
-18.5935101896125));
#4816=CARTESIAN_POINT('Ctrl Pts',(-32.6135681765606,1.50990331349021E-14,
-18.3723738593228));
#4817=CARTESIAN_POINT('Ctrl Pts',(-31.3769595799164,1.24331557212291E-14,
-17.94878125987));
#4818=CARTESIAN_POINT('Ctrl Pts',(-30.1465313472377,1.0222160868584E-14,
-17.504445383288));
#4819=CARTESIAN_POINT('Ctrl Pts',(-28.9220387964689,9.76996261670138E-15,
-17.0391634027186));
#4820=CARTESIAN_POINT('Ctrl Pts',(-28.280905786778,9.53319578130951E-15,
-16.7955460476191));
#4821=CARTESIAN_POINT('Ctrl Pts',(-27.6414002959298,9.73942422296218E-15,
-16.5461855556373));
#4822=CARTESIAN_POINT('Ctrl Pts',(-27.003489002828,1.06581410364015E-14,
-16.2910473999339));
#4823=CARTESIAN_POINT('Ctrl Pts',(-26.9214424596597,1.07763040780476E-14,
-16.2582321732211));
#4824=CARTESIAN_POINT('Ctrl Pts',(-26.8394331456511,1.09599753714691E-14,
-16.2253257263837));
#4825=CARTESIAN_POINT('Ctrl Pts',(-26.7574608858174,1.11022302462516E-14,
-16.1923280234092));
#4826=CARTESIAN_POINT('Ctrl Pts',(-26.6728122570399,1.1249129698721E-14,
-16.158252955633));
#4827=CARTESIAN_POINT('Ctrl Pts',(-26.5882109329397,1.1627230561039E-14,
-16.1240837088094));
#4828=CARTESIAN_POINT('Ctrl Pts',(-26.5036601420706,1.17683640610267E-14,
-16.0898217001875));
#4829=CARTESIAN_POINT('Ctrl Pts',(-25.7442601358659,1.3035966405898E-14,
-15.7820946015686));
#4830=CARTESIAN_POINT('Ctrl Pts',(-24.9888454631677,1.38814835013908E-14,
-15.4668487724091));
#4831=CARTESIAN_POINT('Ctrl Pts',(-24.237230782582,1.46549439250521E-14,
-15.1440887362585));
#4832=CARTESIAN_POINT('Ctrl Pts',(-23.3199064620055,1.55989303531444E-14,
-14.7501693005172));
#4833=CARTESIAN_POINT('Ctrl Pts',(-22.4082668273739,1.50548750441534E-14,
-14.3450675510963));
#4834=CARTESIAN_POINT('Ctrl Pts',(-21.5020580029957,1.62092561595273E-14,
-13.9288016897425));
#4835=CARTESIAN_POINT('Ctrl Pts',(-20.5952669744745,1.73643789201489E-14,
-13.5122683936621));
#4836=CARTESIAN_POINT('Ctrl Pts',(-19.6938847201665,1.57933555484948E-14,
-13.0845414602457));
#4837=CARTESIAN_POINT('Ctrl Pts',(-18.7977536862311,1.62092561595273E-14,
-12.645663195712));
#4838=CARTESIAN_POINT('Ctrl Pts',(-18.3495978945471,1.63062227585341E-14,
-12.4261798515952));
#4839=CARTESIAN_POINT('Ctrl Pts',(-17.9027032335625,1.57814290351876E-14,
-12.2038797705404));
#4840=CARTESIAN_POINT('Ctrl Pts',(-17.4571099588515,1.55431223447522E-14,
-11.9787974606056));
#4841=CARTESIAN_POINT('Ctrl Pts',(-17.0115235519992,1.53048193273002E-14,
-11.7537186198289));
#4842=CARTESIAN_POINT('Ctrl Pts',(-16.5671420195394,1.50389305983309E-14,
-11.5258063384921));
#4843=CARTESIAN_POINT('Ctrl Pts',(-16.1243005352796,1.46549439250521E-14,
-11.2952485538549));
#4844=CARTESIAN_POINT('Ctrl Pts',(-15.2388368853048,1.38871607490214E-14,
-10.8342471690002));
#4845=CARTESIAN_POINT('Ctrl Pts',(-14.359372072549,1.41875053432936E-14,
-10.3626017246681));
#4846=CARTESIAN_POINT('Ctrl Pts',(-13.4855627416189,1.22124532708767E-14,
-9.88029473784141));
#4847=CARTESIAN_POINT('Ctrl Pts',(-12.612368072651,1.02387905054168E-14,
-9.39832701926059));
#4848=CARTESIAN_POINT('Ctrl Pts',(-11.7448449913689,9.99403333149777E-15,
-8.90572622764085));
#4849=CARTESIAN_POINT('Ctrl Pts',(-10.8827350786316,8.65973959207622E-15,
-8.40249416572321));
#4850=CARTESIAN_POINT('Ctrl Pts',(-10.4520277880869,7.99313080727245E-15,
-8.15108107476871));
#4851=CARTESIAN_POINT('Ctrl Pts',(-10.0226717933981,4.28796303457655E-15,
-7.89701412660226));
#4852=CARTESIAN_POINT('Ctrl Pts',(-9.59463597909433,5.32907051820075E-15,
-7.64029160545447));
#4853=CARTESIAN_POINT('Ctrl Pts',(-9.3807251925437,5.84936371158235E-15,
-7.51199459247366));
#4854=CARTESIAN_POINT('Ctrl Pts',(-9.16714413194284,4.59352397126425E-15,
-7.38303433113536));
#4855=CARTESIAN_POINT('Ctrl Pts',(-8.95388898144895,4.66293670342566E-15,
-7.25341048871357));
#4856=CARTESIAN_POINT('Ctrl Pts',(-8.74289238468451,4.73161429561619E-15,
-7.12515947321788));
#4857=CARTESIAN_POINT('Ctrl Pts',(-8.53221483130022,4.37413988992977E-15,
-6.99625885790051));
#4858=CARTESIAN_POINT('Ctrl Pts',(-8.32185266851846,3.99680288865056E-15,
-6.86670824505608));
#4859=CARTESIAN_POINT('',(-16.8843114964558,0.,11.6834750258843));
#4860=CARTESIAN_POINT('Origin',(1.18077271965353,0.,5.54861712757117));
#4861=CARTESIAN_POINT('Ctrl Pts',(-5.24383419181389,1.00000000000006,-6.12586516693238));
#4862=CARTESIAN_POINT('Ctrl Pts',(-5.45552849279514,1.00000000000006,-6.25812980617024));
#4863=CARTESIAN_POINT('Ctrl Pts',(-5.66722279377639,1.00000000000006,-6.39039444540812));
#4864=CARTESIAN_POINT('Ctrl Pts',(-5.98476424524831,1.00000000000006,-6.58879140426484));
#4865=CARTESIAN_POINT('Ctrl Pts',(-6.09061139573891,1.00000000000006,-6.65492372388378));
#4866=CARTESIAN_POINT('Ctrl Pts',(-6.30230569672019,1.00000000000006,-6.78718836312159));
#4867=CARTESIAN_POINT('Ctrl Pts',(-6.40815284721083,1.00000000000006,-6.85332068274051));
#4868=CARTESIAN_POINT('Ctrl Pts',(-6.6198471481921,1.00000000000006,-6.98558532197835));
#4869=CARTESIAN_POINT('Ctrl Pts',(-6.72563063914494,1.00000000000006,-7.05168172755663));
#4870=CARTESIAN_POINT('Ctrl Pts',(-6.88449685418767,1.00000000000006,-7.15093407804603));
#4871=CARTESIAN_POINT('Ctrl Pts',(-6.93738368631082,1.00000000000006,-7.18398126018817));
#4872=CARTESIAN_POINT('Ctrl Pts',(-7.01677641920857,1.00000000000006,-7.23358203087279));
#4873=CARTESIAN_POINT('Ctrl Pts',(-7.04327503493536,1.00000000000006,-7.25013843752416));
#4874=CARTESIAN_POINT('Ctrl Pts',(-7.09612004061923,1.00000000000006,-7.2831569231934));
#4875=CARTESIAN_POINT('Ctrl Pts',(-7.12287909314553,1.00000000000006,-7.29987365377378));
#4876=CARTESIAN_POINT('Ctrl Pts',(-7.20287196849749,1.00000000000006,-7.34979198412591));
#4877=CARTESIAN_POINT('Ctrl Pts',(-7.25627459447878,1.00000000000006,-7.38306454177835));
#4878=CARTESIAN_POINT('Ctrl Pts',(-7.36307503586608,1.00000000000006,-7.44949630138193));
#4879=CARTESIAN_POINT('Ctrl Pts',(-7.41649833999293,1.00000000000006,-7.48267227463444));
#4880=CARTESIAN_POINT('Ctrl Pts',(-7.57683755810601,1.00000000000006,-7.58208037051894));
#4881=CARTESIAN_POINT('Ctrl Pts',(-7.68382277781079,1.00000000000006,-7.64819266931624));
#4882=CARTESIAN_POINT('Ctrl Pts',(-8.00505610385903,1.00000000000006,-7.84604943490794));
#4883=CARTESIAN_POINT('Ctrl Pts',(-8.21958187689062,1.00000000000006,-7.97731377158191));
#4884=CARTESIAN_POINT('Ctrl Pts',(-8.64937624226859,1.00000000000006,-8.23855762413463));
#4885=CARTESIAN_POINT('Ctrl Pts',(-8.86464483463895,1.00000000000006,-8.36853713993857));
#4886=CARTESIAN_POINT('Ctrl Pts',(-9.51156841532699,1.00000000000005,-8.75654171121627));
#4887=CARTESIAN_POINT('Ctrl Pts',(-9.94434120352226,1.00000000000006,-9.01263280045349));
#4888=CARTESIAN_POINT('Ctrl Pts',(-11.2471595199954,1.00000000000006,-9.77311581787846));
#4889=CARTESIAN_POINT('Ctrl Pts',(-12.1217049333607,1.00000000000006,-10.2697176721681));
#4890=CARTESIAN_POINT('Ctrl Pts',(-13.8829505118507,1.00000000000006,-11.2418531471041));
#4891=CARTESIAN_POINT('Ctrl Pts',(-14.7696264087533,1.00000000000006,-11.7173731122773));
#4892=CARTESIAN_POINT('Ctrl Pts',(-16.1089470909339,1.00000000000006,-12.4146673382703));
#4893=CARTESIAN_POINT('Ctrl Pts',(-16.5569782215825,1.00000000000006,-12.6444517294623));
#4894=CARTESIAN_POINT('Ctrl Pts',(-17.4554954883835,1.00000000000006,-13.0983193110247));
#4895=CARTESIAN_POINT('Ctrl Pts',(-17.9060788716974,1.00000000000006,-13.3224542098502));
#4896=CARTESIAN_POINT('Ctrl Pts',(-19.2616031097108,1.00000000000006,-13.9863193171645));
#4897=CARTESIAN_POINT('Ctrl Pts',(-20.1705291712439,1.00000000000006,-14.4176206450584));
#4898=CARTESIAN_POINT('Ctrl Pts',(-21.9987526788008,1.00000000000006,-15.2574127694115));
#4899=CARTESIAN_POINT('Ctrl Pts',(-22.9180793896471,1.00000000000006,-15.6659188375137));
#4900=CARTESIAN_POINT('Ctrl Pts',(-24.7672228950628,1.00000000000006,-16.4599821261938));
#4901=CARTESIAN_POINT('Ctrl Pts',(-25.6970148613833,1.00000000000006,-16.8455293489637));
#4902=CARTESIAN_POINT('Ctrl Pts',(-28.5023646567929,1.00000000000006,-17.9675533325283));
#4903=CARTESIAN_POINT('Ctrl Pts',(-30.3883028921554,1.00000000000006,-18.6671643210093));
#4904=CARTESIAN_POINT('Ctrl Pts',(-34.1907153053487,1.00000000000006,-19.9696570897424));
#4905=CARTESIAN_POINT('Ctrl Pts',(-36.1073577041579,1.00000000000006,-20.5725959425394));
#4906=CARTESIAN_POINT('Ctrl Pts',(-39.0050100165848,1.00000000000006,-21.4047438218093));
#4907=CARTESIAN_POINT('Ctrl Pts',(-39.9748094572256,1.00000000000006,-21.6701144864535));
#4908=CARTESIAN_POINT('Ctrl Pts',(-41.4350320957616,1.00000000000006,-22.0501116296716));
#4909=CARTESIAN_POINT('Ctrl Pts',(-41.922768748648,1.00000000000006,-22.173784814017));
#4910=CARTESIAN_POINT('Ctrl Pts',(-42.900075718841,1.00000000000006,-22.4151175190879));
#4911=CARTESIAN_POINT('Ctrl Pts',(-43.3897554961037,1.00000000000006,-22.5328007101756));
#4912=CARTESIAN_POINT('Ctrl Pts',(-44.370090732942,1.00000000000006,-22.7619636311583));
#4913=CARTESIAN_POINT('Ctrl Pts',(-44.8609173199214,1.00000000000006,-22.8734864251602));
#4914=CARTESIAN_POINT('Ctrl Pts',(-45.5980622108449,1.00000000000006,-23.0361857718529));
#4915=CARTESIAN_POINT('Ctrl Pts',(-45.8439323102181,1.00000000000006,-23.0896558259346));
#4916=CARTESIAN_POINT('Ctrl Pts',(-46.3359817814183,1.00000000000006,-23.19507356367));
#4917=CARTESIAN_POINT('Ctrl Pts',(-46.5821611532186,1.00000000000006,-23.2470212473572));
#4918=CARTESIAN_POINT('Ctrl Pts',(-46.9516614198392,1.00000000000006,-23.3238038024982));
#4919=CARTESIAN_POINT('Ctrl Pts',(-47.0748667102372,1.00000000000006,-23.349208159078));
#4920=CARTESIAN_POINT('Ctrl Pts',(-47.2597323553301,1.00000000000006,-23.3870303014924));
#4921=CARTESIAN_POINT('Ctrl Pts',(-47.321363855279,1.00000000000006,-23.3995902835508));
#4922=CARTESIAN_POINT('Ctrl Pts',(-47.444646076246,1.00000000000006,-23.4246155084937));
#4923=CARTESIAN_POINT('Ctrl Pts',(-47.5063283010135,1.00000000000006,-23.4370863095799));
#4924=CARTESIAN_POINT('Ctrl Pts',(-47.5987715311571,1.00000000000006,-23.4557048259362));
#4925=CARTESIAN_POINT('Ctrl Pts',(-47.6297134045,1.00000000000006,-23.4619201822993));
#4926=CARTESIAN_POINT('Ctrl Pts',(-47.6907845360928,1.00000000000006,-23.4741826558094));
#4927=CARTESIAN_POINT('Ctrl Pts',(-47.7214121565107,1.00000000000006,-23.4803327329731));
#4928=CARTESIAN_POINT('Ctrl Pts',(-47.813167153602,1.00000000000006,-23.498760940644));
#4929=CARTESIAN_POINT('Ctrl Pts',(-47.8743280692006,1.00000000000006,-23.5110408686088));
#4930=CARTESIAN_POINT('Ctrl Pts',(-47.9966589828603,1.00000000000006,-23.5356062683543));
#4931=CARTESIAN_POINT('Ctrl Pts',(-48.05782443969,1.00000000000006,-23.5478889682269));
#4932=CARTESIAN_POINT('Ctrl Pts',(-48.1801553533496,1.00000000000006,-23.5724543679724));
#4933=CARTESIAN_POINT('Ctrl Pts',(-48.2413208101794,1.00000000000006,-23.584737067845));
#4934=CARTESIAN_POINT('Ctrl Pts',(-48.4248171806689,1.00000000000006,-23.6215851674632));
#4935=CARTESIAN_POINT('Ctrl Pts',(-48.5471480943282,1.00000000000006,-23.6461505672086));
#4936=CARTESIAN_POINT('Ctrl Pts',(-48.7918099216474,1.00000000000006,-23.6952813666994));
#4937=CARTESIAN_POINT('Ctrl Pts',(-48.914140835307,1.00000000000006,-23.7198467664448));
#4938=CARTESIAN_POINT('Ctrl Pts',(-49.2811335762858,1.00000000000006,-23.793542965681));
#4939=CARTESIAN_POINT('Ctrl Pts',(-49.525795403605,1.00000000000006,-23.8426737651719));
#4940=CARTESIAN_POINT('Ctrl Pts',(-49.770457230924,1.00000000000006,-23.8918045646627));
#4941=CARTESIAN_POINT('Ctrl Pts',(-5.77370550858122,0.,-5.27778711175859));
#4942=CARTESIAN_POINT('Ctrl Pts',(-5.9853998095625,0.,-5.41005175099646));
#4943=CARTESIAN_POINT('Ctrl Pts',(-6.19709411054381,0.,-5.54231639023431));
#4944=CARTESIAN_POINT('Ctrl Pts',(-6.51463556201566,0.,-5.74071334909106));
#4945=CARTESIAN_POINT('Ctrl Pts',(-6.62048271250629,0.,-5.80684566871));
#4946=CARTESIAN_POINT('Ctrl Pts',(-6.83217701348755,0.,-5.93911030794779));
#4947=CARTESIAN_POINT('Ctrl Pts',(-6.93802416397819,0.,-6.00524262756673));
#4948=CARTESIAN_POINT('Ctrl Pts',(-7.14971846495949,0.,-6.13750726680458));
#4949=CARTESIAN_POINT('Ctrl Pts',(-7.25556400272244,0.,-6.20364240870763));
#4950=CARTESIAN_POINT('Ctrl Pts',(-7.41433714754994,0.,-6.30283665470982));
#4951=CARTESIAN_POINT('Ctrl Pts',(-7.46725906024219,0.,-6.33590572399238));
#4952=CARTESIAN_POINT('Ctrl Pts',(-7.54664570739394,0.,-6.38550271620998));
#4953=CARTESIAN_POINT('Ctrl Pts',(-7.57310736259635,0.,-6.40203602780547));
#4954=CARTESIAN_POINT('Ctrl Pts',(-7.62603034649297,0.,-6.43510322256449));
#4955=CARTESIAN_POINT('Ctrl Pts',(-7.65249300217831,0.,-6.45163478324257));
#4956=CARTESIAN_POINT('Ctrl Pts',(-7.73190363272615,-8.67361737988404E-16,
-6.50118980170777));
#4957=CARTESIAN_POINT('Ctrl Pts',(-7.78486602535483,8.67361737988404E-16,
-6.53418802672631));
#4958=CARTESIAN_POINT('Ctrl Pts',(-7.8908369143435,-8.67361737988404E-16,
-6.60010379009612));
#4959=CARTESIAN_POINT('Ctrl Pts',(-7.94384505715716,8.67361737988404E-16,
-6.63302194717649));
#4960=CARTESIAN_POINT('Ctrl Pts',(-8.1029376375198,-8.67361737988404E-16,
-6.73165714491127));
#4961=CARTESIAN_POINT('Ctrl Pts',(-8.20909022696902,0.,-6.79725491209686));
#4962=CARTESIAN_POINT('Ctrl Pts',(-8.52782105955695,0.,-6.99357032060786));
#4963=CARTESIAN_POINT('Ctrl Pts',(-8.74067236655293,0.,-7.12381006955848));
#4964=CARTESIAN_POINT('Ctrl Pts',(-9.16710559634496,-8.67361737988404E-16,
-7.38301090786864));
#4965=CARTESIAN_POINT('Ctrl Pts',(-9.38068751917746,0.,-7.51197199716448));
#4966=CARTESIAN_POINT('Ctrl Pts',(-10.0225328989281,-2.60208521396521E-15,
-7.89693082203444));
#4967=CARTESIAN_POINT('Ctrl Pts',(-10.4518959613416,0.,-8.15100412466771));
#4968=CARTESIAN_POINT('Ctrl Pts',(-11.7444133132118,0.,-8.90547424783421));
#4969=CARTESIAN_POINT('Ctrl Pts',(-12.6119956637783,-8.67361737988404E-16,
-9.39812146480502));
#4970=CARTESIAN_POINT('Ctrl Pts',(-14.3591298194595,8.67361737988404E-16,
-10.3624680108778));
#4971=CARTESIAN_POINT('Ctrl Pts',(-15.2386575500661,0.,-10.8341538011997));
#4972=CARTESIAN_POINT('Ctrl Pts',(-16.5671220278863,0.,-11.5257959301825));
#4973=CARTESIAN_POINT('Ctrl Pts',(-17.0115117764597,0.,-11.7537126716564));
#4974=CARTESIAN_POINT('Ctrl Pts',(-17.9027081412433,0.,-12.2038822495548));
#4975=CARTESIAN_POINT('Ctrl Pts',(-18.3496112197363,0.,-12.4261863775782));
#4976=CARTESIAN_POINT('Ctrl Pts',(-19.6940386192206,-8.67361737988404E-16,
-13.0846168319795));
#4977=CARTESIAN_POINT('Ctrl Pts',(-20.5954904839877,8.67361737988404E-16,
-13.5123710624704));
#4978=CARTESIAN_POINT('Ctrl Pts',(-22.4086255220037,-8.67361737988404E-16,
-14.3452323170145));
#4979=CARTESIAN_POINT('Ctrl Pts',(-23.3203377275709,0.,-14.7503544955288));
#4980=CARTESIAN_POINT('Ctrl Pts',(-25.1541238375931,0.,-15.5378229769881));
#4981=CARTESIAN_POINT('Ctrl Pts',(-26.0761731394061,0.,-15.9201593756798));
#4982=CARTESIAN_POINT('Ctrl Pts',(-28.8581207296717,0.,-17.0328234484422));
#4983=CARTESIAN_POINT('Ctrl Pts',(-30.7282718716483,0.,-17.726577311649));
#4984=CARTESIAN_POINT('Ctrl Pts',(-34.4988644814729,0.,-19.0181704069966));
#4985=CARTESIAN_POINT('Ctrl Pts',(-36.3994730456328,0.,-19.6160663145302));
#4986=CARTESIAN_POINT('Ctrl Pts',(-39.2729851137603,0.,-20.4412815926138));
#4987=CARTESIAN_POINT('Ctrl Pts',(-40.2347218365622,1.73472347597681E-15,
-20.7044462959577));
#4988=CARTESIAN_POINT('Ctrl Pts',(-41.6828409388869,0.,-21.0812937073895));
#4989=CARTESIAN_POINT('Ctrl Pts',(-42.1665408867303,8.67361737988404E-16,
-21.2039433661147));
#4990=CARTESIAN_POINT('Ctrl Pts',(-43.1357732858097,0.,-21.4432821653729));
#4991=CARTESIAN_POINT('Ctrl Pts',(-43.6214143011738,0.,-21.5599947826799));
#4992=CARTESIAN_POINT('Ctrl Pts',(-44.5936798235137,0.,-21.7872713292545));
#4993=CARTESIAN_POINT('Ctrl Pts',(-45.0804740425724,0.,-21.8978779663177));
#4994=CARTESIAN_POINT('Ctrl Pts',(-45.8115761744865,0.,-22.0592435820542));
#4995=CARTESIAN_POINT('Ctrl Pts',(-46.0554329505363,0.,-22.1122758004251));
#4996=CARTESIAN_POINT('Ctrl Pts',(-46.5434578674449,0.,-22.2168313089879));
#4997=CARTESIAN_POINT('Ctrl Pts',(-46.7876260082956,0.,-22.268354599221));
#4998=CARTESIAN_POINT('Ctrl Pts',(-47.1541111707643,0.,-22.3445106124556));
#4999=CARTESIAN_POINT('Ctrl Pts',(-47.2763117168066,0.,-22.3697077964145));
#5000=CARTESIAN_POINT('Ctrl Pts',(-47.4596707023514,0.,-22.4072216874391));
#5001=CARTESIAN_POINT('Ctrl Pts',(-47.5208000586142,0.,-22.4196793369561));
#5002=CARTESIAN_POINT('Ctrl Pts',(-47.6430781480945,0.,-22.4445007318891));
#5003=CARTESIAN_POINT('Ctrl Pts',(-47.7042270322544,0.,-22.4568637457667));
#5004=CARTESIAN_POINT('Ctrl Pts',(-47.7959644294841,0.,-22.4753400762447));
#5005=CARTESIAN_POINT('Ctrl Pts',(-47.8265467872086,0.,-22.4814832225577));
#5006=CARTESIAN_POINT('Ctrl Pts',(-47.8877124965496,0.,-22.493764698779));
#5007=CARTESIAN_POINT('Ctrl Pts',(-47.9182952814496,0.,-22.4999057748181));
#5008=CARTESIAN_POINT('Ctrl Pts',(-48.0100429184723,0.,-22.518332481796));
#5009=CARTESIAN_POINT('Ctrl Pts',(-48.0712087407834,0.,-22.5306134102228));
#5010=CARTESIAN_POINT('Ctrl Pts',(-48.193539654443,0.,-22.5551788099683));
#5011=CARTESIAN_POINT('Ctrl Pts',(-48.2547051112727,0.,-22.5674615098409));
#5012=CARTESIAN_POINT('Ctrl Pts',(-48.3770360249324,0.,-22.5920269095863));
#5013=CARTESIAN_POINT('Ctrl Pts',(-48.4382014817621,0.,-22.604309609459));
#5014=CARTESIAN_POINT('Ctrl Pts',(-48.6216978522517,0.,-22.6411577090772));
#5015=CARTESIAN_POINT('Ctrl Pts',(-48.744028765911,0.,-22.6657231088225));
#5016=CARTESIAN_POINT('Ctrl Pts',(-48.9886905932302,0.,-22.7148539083134));
#5017=CARTESIAN_POINT('Ctrl Pts',(-49.1110215068898,0.,-22.7394193080588));
#5018=CARTESIAN_POINT('Ctrl Pts',(-49.4780142478686,0.,-22.813115507295));
#5019=CARTESIAN_POINT('Ctrl Pts',(-49.7226760751877,0.,-22.8622463067859));
#5020=CARTESIAN_POINT('Ctrl Pts',(-49.9673379025068,0.,-22.9113771062766));
#12115=UNCERTAINTY_MEASURE_WITH_UNIT(LENGTH_MEASURE(0.01),#12138,
'DISTANCE_ACCURACY_VALUE',
'Maximum model space distance between geometric entities at asserted c
onnectivities');
#12123=UNCERTAINTY_MEASURE_WITH_UNIT(LENGTH_MEASURE(0.01),#12138,
'DISTANCE_ACCURACY_VALUE',
'Maximum model space distance between geometric entities at asserted c
onnectivities');
#12129=(
GEOMETRIC_REPRESENTATION_CONTEXT(3)
GLOBAL_UNCERTAINTY_ASSIGNED_CONTEXT((#12115))
GLOBAL_UNIT_ASSIGNED_CONTEXT((#12138,#12140,#12141))
REPRESENTATION_CONTEXT('','3D')
);
#12137=(
GEOMETRIC_REPRESENTATION_CONTEXT(3)
GLOBAL_UNCERTAINTY_ASSIGNED_CONTEXT((#12123))
GLOBAL_UNIT_ASSIGNED_CONTEXT((#12138,#12140,#12141))
REPRESENTATION_CONTEXT('','3D')
);
#12138=(
LENGTH_UNIT()
NAMED_UNIT(*)
SI_UNIT(.MILLI.,.METRE.)
);
#12140=(
NAMED_UNIT(*)
PLANE_ANGLE_UNIT()
SI_UNIT($,.RADIAN.)
);
#12141=(
NAMED_UNIT(*)
SI_UNIT($,.STERADIAN.)
SOLID_ANGLE_UNIT()
);
#12147=SHAPE_DEFINITION_REPRESENTATION(#12160,#12188);
#12160=PRODUCT_DEFINITION_SHAPE('',$,#12202);
#12188=SHAPE_REPRESENTATION('',(#2014),#12129);
#12196=PRODUCT_DEFINITION_CONTEXT('part definition',#12237,'design');
#12202=PRODUCT_DEFINITION('casy 1','Blade_1',#12215,#12196);
#12215=PRODUCT_DEFINITION_FORMATION('',$,#12244);
#12237=APPLICATION_CONTEXT(
'Core Data for Automotive Mechanical Design Process');
#12238=PRODUCT_CONTEXT('part definition',#12237,'mechanical');
#12244=PRODUCT('casy 1','Blade_1',$,(#12238));
#12253=PRESENTATION_STYLE_ASSIGNMENT((#12255));
#12255=SURFACE_STYLE_USAGE(.BOTH.,#12257);
#12257=SURFACE_SIDE_STYLE('',(#12259));
#12259=SURFACE_STYLE_FILL_AREA(#12261);
#12261=FILL_AREA_STYLE('Opaque(23,69,131)',(#12263));
#12263=FILL_AREA_STYLE_COLOUR('Opaque(23,69,131)',#12265);
#12265=COLOUR_RGB('Opaque(23,69,131)',0.0901960784313725,0.270588235294118,
0.513725490196078);
ENDSEC;
END-ISO-10303-21;
